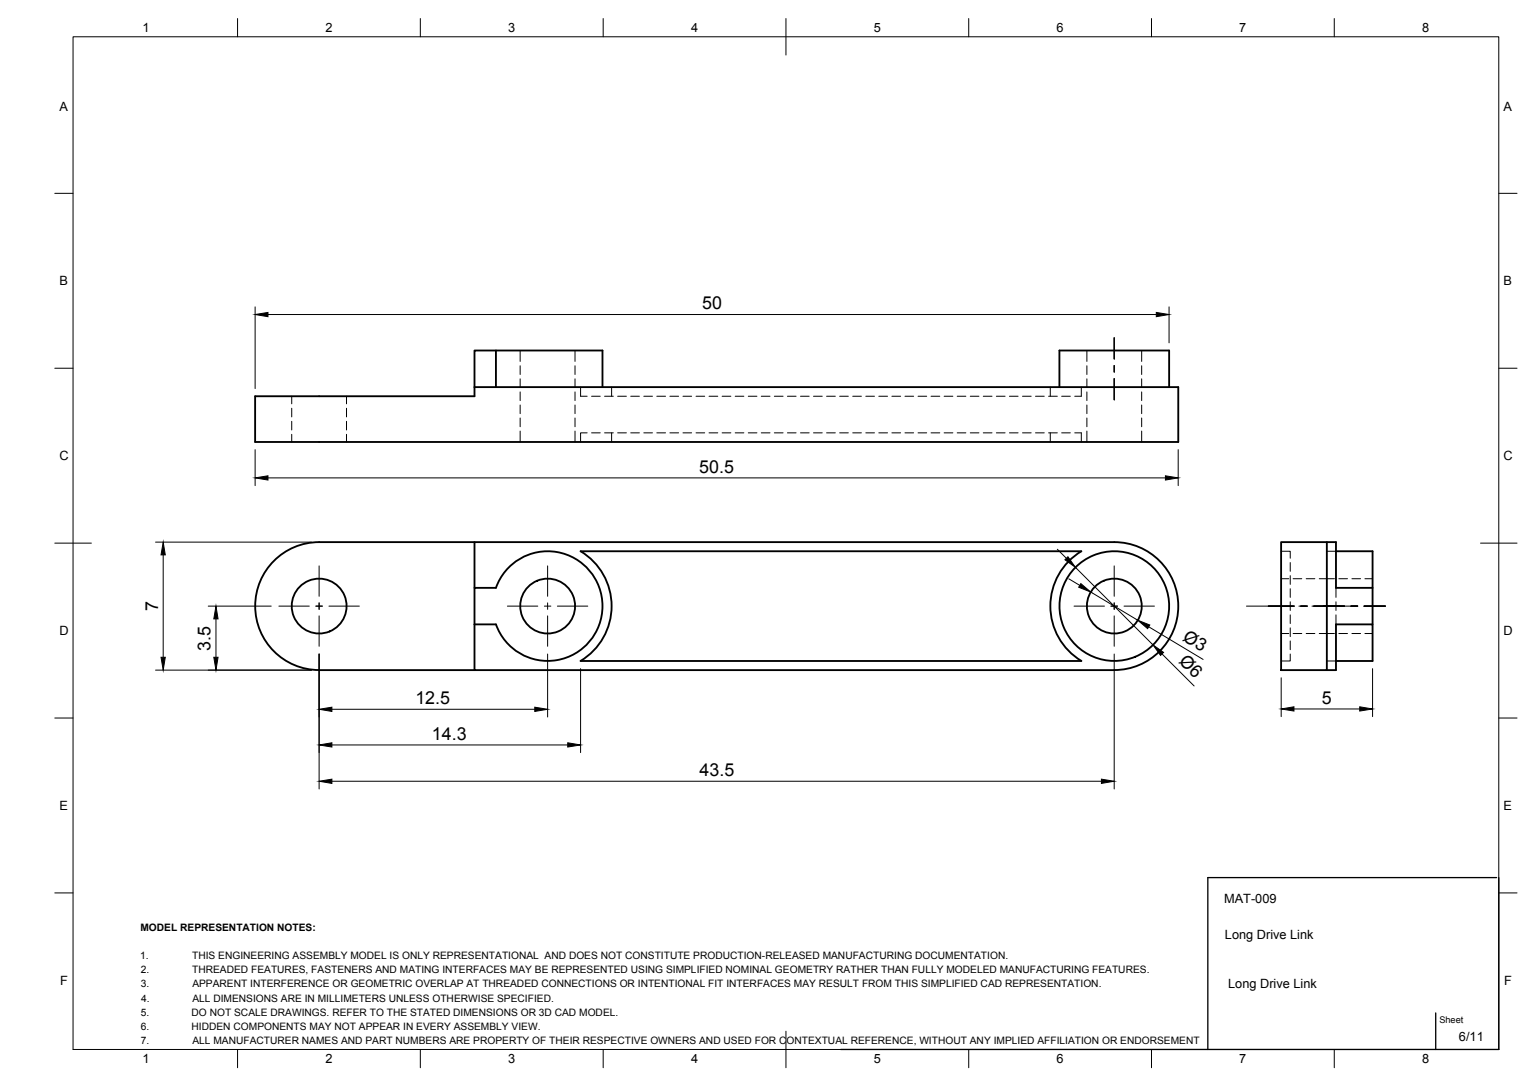
ISO-10303-21;
HEADER;
/* Generated by software containing ST-Developer
 * from STEP Tools, Inc. (www.steptools.com) 
 */

FILE_DESCRIPTION(
/* description */ ('STEP AP214'),
/* implementation_level */ '2;1');

FILE_NAME(
/* name */ 'Long Drive Link.step',
/* time_stamp */ '2026-11-14T05:43:09-08:00',
/* author */ (''),
/* organization */ (''),
/* preprocessor_version */ 'ST-DEVELOPER v20.2',
/* originating_system */ 'Autodesk Translation Framework v15.17.0.0',
/* authorisation */ '');

FILE_SCHEMA (('AUTOMOTIVE_DESIGN { 1 0 10303 214 3 1 1 }'));
ENDSEC;

DATA;
#10=MECHANICAL_DESIGN_GEOMETRIC_PRESENTATION_REPRESENTATION('',(#148),#11933);
#130=SHAPE_REPRESENTATION_RELATIONSHIP('SRR','None',#11990,#139);
#139=ADVANCED_BREP_SHAPE_REPRESENTATION('',(#157),#11926);
#148=STYLED_ITEM('',(#12043),#157);
#157=MANIFOLD_SOLID_BREP('Body1',#6645);
#183=FACE_BOUND('',#748,.T.);
#184=FACE_BOUND('',#750,.T.);
#185=FACE_BOUND('',#751,.T.);
#186=FACE_BOUND('',#753,.T.);
#187=FACE_BOUND('',#754,.T.);
#188=FACE_BOUND('',#755,.T.);
#189=FACE_BOUND('',#756,.T.);
#190=FACE_BOUND('',#773,.T.);
#191=FACE_BOUND('',#775,.T.);
#235=PLANE('',#6871);
#236=PLANE('',#6872);
#237=PLANE('',#6876);
#238=PLANE('',#6879);
#239=PLANE('',#6881);
#240=PLANE('',#6884);
#241=PLANE('',#6885);
#242=PLANE('',#6886);
#243=PLANE('',#6887);
#244=PLANE('',#6890);
#245=PLANE('',#6891);
#246=PLANE('',#6892);
#247=PLANE('',#6895);
#248=PLANE('',#6896);
#249=PLANE('',#6897);
#250=PLANE('',#6898);
#367=FACE_OUTER_BOUND('',#740,.T.);
#368=FACE_OUTER_BOUND('',#741,.T.);
#369=FACE_OUTER_BOUND('',#742,.T.);
#370=FACE_OUTER_BOUND('',#743,.T.);
#371=FACE_OUTER_BOUND('',#744,.T.);
#372=FACE_OUTER_BOUND('',#745,.T.);
#373=FACE_OUTER_BOUND('',#746,.T.);
#374=FACE_OUTER_BOUND('',#747,.T.);
#375=FACE_OUTER_BOUND('',#749,.T.);
#376=FACE_OUTER_BOUND('',#752,.T.);
#377=FACE_OUTER_BOUND('',#757,.T.);
#378=FACE_OUTER_BOUND('',#758,.T.);
#379=FACE_OUTER_BOUND('',#759,.T.);
#380=FACE_OUTER_BOUND('',#760,.T.);
#381=FACE_OUTER_BOUND('',#761,.T.);
#382=FACE_OUTER_BOUND('',#762,.T.);
#383=FACE_OUTER_BOUND('',#763,.T.);
#384=FACE_OUTER_BOUND('',#764,.T.);
#385=FACE_OUTER_BOUND('',#765,.T.);
#386=FACE_OUTER_BOUND('',#766,.T.);
#387=FACE_OUTER_BOUND('',#767,.T.);
#388=FACE_OUTER_BOUND('',#768,.T.);
#389=FACE_OUTER_BOUND('',#769,.T.);
#390=FACE_OUTER_BOUND('',#770,.T.);
#391=FACE_OUTER_BOUND('',#771,.T.);
#392=FACE_OUTER_BOUND('',#772,.T.);
#393=FACE_OUTER_BOUND('',#774,.T.);
#740=EDGE_LOOP('',(#4354,#4355,#4356,#4357));
#741=EDGE_LOOP('',(#4358,#4359,#4360,#4361));
#742=EDGE_LOOP('',(#4362,#4363,#4364,#4365));
#743=EDGE_LOOP('',(#4366,#4367,#4368,#4369));
#744=EDGE_LOOP('',(#4370,#4371,#4372,#4373));
#745=EDGE_LOOP('',(#4374,#4375,#4376,#4377));
#746=EDGE_LOOP('',(#4378,#4379,#4380,#4381));
#747=EDGE_LOOP('',(#4382,#4383,#4384,#4385));
#748=EDGE_LOOP('',(#4386));
#749=EDGE_LOOP('',(#4387,#4388,#4389,#4390,#4391,#4392,#4393,#4394));
#750=EDGE_LOOP('',(#4395,#4396,#4397,#4398));
#751=EDGE_LOOP('',(#4399));
#752=EDGE_LOOP('',(#4400,#4401,#4402,#4403));
#753=EDGE_LOOP('',(#4404));
#754=EDGE_LOOP('',(#4405,#4406,#4407,#4408));
#755=EDGE_LOOP('',(#4409));
#756=EDGE_LOOP('',(#4410));
#757=EDGE_LOOP('',(#4411,#4412,#4413,#4414,#4415,#4416));
#758=EDGE_LOOP('',(#4417,#4418,#4419,#4420));
#759=EDGE_LOOP('',(#4421,#4422,#4423,#4424,#4425,#4426));
#760=EDGE_LOOP('',(#4427,#4428,#4429,#4430));
#761=EDGE_LOOP('',(#4431,#4432,#4433,#4434));
#762=EDGE_LOOP('',(#4435,#4436,#4437,#4438));
#763=EDGE_LOOP('',(#4439,#4440,#4441,#4442));
#764=EDGE_LOOP('',(#4443,#4444,#4445,#4446));
#765=EDGE_LOOP('',(#4447,#4448,#4449,#4450));
#766=EDGE_LOOP('',(#4451,#4452,#4453,#4454));
#767=EDGE_LOOP('',(#4455,#4456,#4457,#4458));
#768=EDGE_LOOP('',(#4459,#4460,#4461,#4462));
#769=EDGE_LOOP('',(#4463,#4464,#4465,#4466));
#770=EDGE_LOOP('',(#4467,#4468,#4469,#4470));
#771=EDGE_LOOP('',(#4471,#4472,#4473,#4474,#4475,#4476,#4477,#4478));
#772=EDGE_LOOP('',(#4479,#4480,#4481,#4482));
#773=EDGE_LOOP('',(#4483));
#774=EDGE_LOOP('',(#4484));
#775=EDGE_LOOP('',(#4485));
#1147=LINE('',#10165,#1609);
#1148=LINE('',#10172,#1610);
#1149=LINE('',#10175,#1611);
#1150=LINE('',#10180,#1612);
#1151=LINE('',#10187,#1613);
#1152=LINE('',#10190,#1614);
#1153=LINE('',#10196,#1615);
#1154=LINE('',#10199,#1616);
#1155=LINE('',#10204,#1617);
#1156=LINE('',#10210,#1618);
#1157=LINE('',#10214,#1619);
#1158=LINE('',#10216,#1620);
#1159=LINE('',#10217,#1621);
#1160=LINE('',#10223,#1622);
#1161=LINE('',#10225,#1623);
#1162=LINE('',#10227,#1624);
#1163=LINE('',#10231,#1625);
#1164=LINE('',#10233,#1626);
#1165=LINE('',#10234,#1627);
#1166=LINE('',#10238,#1628);
#1167=LINE('',#10239,#1629);
#1168=LINE('',#10242,#1630);
#1169=LINE('',#10244,#1631);
#1170=LINE('',#10247,#1632);
#1171=LINE('',#10250,#1633);
#1172=LINE('',#10252,#1634);
#1173=LINE('',#10253,#1635);
#1174=LINE('',#10255,#1636);
#1175=LINE('',#10257,#1637);
#1176=LINE('',#10260,#1638);
#1177=LINE('',#10263,#1639);
#1178=LINE('',#10265,#1640);
#1179=LINE('',#10267,#1641);
#1180=LINE('',#10271,#1642);
#1181=LINE('',#10272,#1643);
#1182=LINE('',#10276,#1644);
#1183=LINE('',#10278,#1645);
#1184=LINE('',#10282,#1646);
#1185=LINE('',#10284,#1647);
#1186=LINE('',#10285,#1648);
#1187=LINE('',#10288,#1649);
#1188=LINE('',#10292,#1650);
#1189=LINE('',#10293,#1651);
#1190=LINE('',#10295,#1652);
#1609=VECTOR('',#7925,1.5);
#1610=VECTOR('',#7932,1000.);
#1611=VECTOR('',#7935,1000.);
#1612=VECTOR('',#7940,3.);
#1613=VECTOR('',#7947,1000.);
#1614=VECTOR('',#7950,1000.);
#1615=VECTOR('',#7955,1000.);
#1616=VECTOR('',#7958,1000.);
#1617=VECTOR('',#7963,1.5);
#1618=VECTOR('',#7970,1.5);
#1619=VECTOR('',#7975,1000.);
#1620=VECTOR('',#7976,1000.);
#1621=VECTOR('',#7977,1000.);
#1622=VECTOR('',#7982,1000.);
#1623=VECTOR('',#7983,1000.);
#1624=VECTOR('',#7984,1000.);
#1625=VECTOR('',#7987,1000.);
#1626=VECTOR('',#7988,1000.);
#1627=VECTOR('',#7989,1000.);
#1628=VECTOR('',#7992,1000.);
#1629=VECTOR('',#7993,1000.);
#1630=VECTOR('',#7996,1000.);
#1631=VECTOR('',#7997,1000.);
#1632=VECTOR('',#8000,1000.);
#1633=VECTOR('',#8003,1000.);
#1634=VECTOR('',#8006,1000.);
#1635=VECTOR('',#8007,1000.);
#1636=VECTOR('',#8010,1000.);
#1637=VECTOR('',#8013,1000.);
#1638=VECTOR('',#8016,1000.);
#1639=VECTOR('',#8019,1000.);
#1640=VECTOR('',#8022,1000.);
#1641=VECTOR('',#8025,1000.);
#1642=VECTOR('',#8030,1000.);
#1643=VECTOR('',#8031,1000.);
#1644=VECTOR('',#8036,1000.);
#1645=VECTOR('',#8039,1000.);
#1646=VECTOR('',#8044,1000.);
#1647=VECTOR('',#8045,1000.);
#1648=VECTOR('',#8046,1000.);
#1649=VECTOR('',#8049,1000.);
#1650=VECTOR('',#8054,1000.);
#1651=VECTOR('',#8055,1000.);
#1652=VECTOR('',#8058,1000.);
#2042=CIRCLE('',#6851,1.5);
#2043=CIRCLE('',#6852,1.5);
#2044=CIRCLE('',#6854,3.5);
#2045=CIRCLE('',#6855,3.5);
#2046=CIRCLE('',#6857,3.);
#2047=CIRCLE('',#6858,3.);
#2048=CIRCLE('',#6860,3.5);
#2049=CIRCLE('',#6861,3.5);
#2050=CIRCLE('',#6863,3.5);
#2051=CIRCLE('',#6864,3.5);
#2052=CIRCLE('',#6866,1.5);
#2053=CIRCLE('',#6867,1.5);
#2054=CIRCLE('',#6869,1.5);
#2055=CIRCLE('',#6870,1.5);
#2056=CIRCLE('',#6873,3.);
#2057=CIRCLE('',#6874,3.5);
#2058=CIRCLE('',#6875,3.5);
#2059=CIRCLE('',#6877,3.5);
#2060=CIRCLE('',#6878,3.5);
#2061=CIRCLE('',#6883,3.5);
#2062=CIRCLE('',#6889,3.5);
#2063=CIRCLE('',#6894,3.);
#2581=VERTEX_POINT('',#10162);
#2582=VERTEX_POINT('',#10164);
#2583=VERTEX_POINT('',#10168);
#2584=VERTEX_POINT('',#10169);
#2585=VERTEX_POINT('',#10171);
#2586=VERTEX_POINT('',#10173);
#2587=VERTEX_POINT('',#10177);
#2588=VERTEX_POINT('',#10179);
#2589=VERTEX_POINT('',#10183);
#2590=VERTEX_POINT('',#10184);
#2591=VERTEX_POINT('',#10186);
#2592=VERTEX_POINT('',#10188);
#2593=VERTEX_POINT('',#10192);
#2594=VERTEX_POINT('',#10193);
#2595=VERTEX_POINT('',#10195);
#2596=VERTEX_POINT('',#10197);
#2597=VERTEX_POINT('',#10201);
#2598=VERTEX_POINT('',#10203);
#2599=VERTEX_POINT('',#10207);
#2600=VERTEX_POINT('',#10209);
#2601=VERTEX_POINT('',#10213);
#2602=VERTEX_POINT('',#10215);
#2603=VERTEX_POINT('',#10219);
#2604=VERTEX_POINT('',#10220);
#2605=VERTEX_POINT('',#10222);
#2606=VERTEX_POINT('',#10224);
#2607=VERTEX_POINT('',#10226);
#2608=VERTEX_POINT('',#10228);
#2609=VERTEX_POINT('',#10230);
#2610=VERTEX_POINT('',#10232);
#2611=VERTEX_POINT('',#10235);
#2612=VERTEX_POINT('',#10236);
#2613=VERTEX_POINT('',#10241);
#2614=VERTEX_POINT('',#10243);
#2615=VERTEX_POINT('',#10246);
#2616=VERTEX_POINT('',#10248);
#2617=VERTEX_POINT('',#10259);
#2618=VERTEX_POINT('',#10261);
#2619=VERTEX_POINT('',#10270);
#2620=VERTEX_POINT('',#10274);
#2621=VERTEX_POINT('',#10281);
#2622=VERTEX_POINT('',#10283);
#2623=VERTEX_POINT('',#10287);
#2624=VERTEX_POINT('',#10291);
#3266=EDGE_CURVE('',#2581,#2581,#2042,.T.);
#3267=EDGE_CURVE('',#2581,#2582,#1147,.T.);
#3268=EDGE_CURVE('',#2582,#2582,#2043,.T.);
#3269=EDGE_CURVE('',#2583,#2584,#2044,.T.);
#3270=EDGE_CURVE('',#2583,#2585,#1148,.T.);
#3271=EDGE_CURVE('',#2585,#2586,#2045,.T.);
#3272=EDGE_CURVE('',#2584,#2586,#1149,.T.);
#3273=EDGE_CURVE('',#2587,#2587,#2046,.T.);
#3274=EDGE_CURVE('',#2587,#2588,#1150,.T.);
#3275=EDGE_CURVE('',#2588,#2588,#2047,.T.);
#3276=EDGE_CURVE('',#2589,#2590,#2048,.T.);
#3277=EDGE_CURVE('',#2590,#2591,#1151,.T.);
#3278=EDGE_CURVE('',#2592,#2591,#2049,.T.);
#3279=EDGE_CURVE('',#2589,#2592,#1152,.T.);
#3280=EDGE_CURVE('',#2593,#2594,#2050,.T.);
#3281=EDGE_CURVE('',#2593,#2595,#1153,.T.);
#3282=EDGE_CURVE('',#2595,#2596,#2051,.T.);
#3283=EDGE_CURVE('',#2594,#2596,#1154,.T.);
#3284=EDGE_CURVE('',#2597,#2597,#2052,.T.);
#3285=EDGE_CURVE('',#2597,#2598,#1155,.T.);
#3286=EDGE_CURVE('',#2598,#2598,#2053,.T.);
#3287=EDGE_CURVE('',#2599,#2599,#2054,.T.);
#3288=EDGE_CURVE('',#2599,#2600,#1156,.T.);
#3289=EDGE_CURVE('',#2600,#2600,#2055,.T.);
#3290=EDGE_CURVE('',#2584,#2601,#1157,.T.);
#3291=EDGE_CURVE('',#2602,#2601,#1158,.T.);
#3292=EDGE_CURVE('',#2602,#2583,#1159,.T.);
#3293=EDGE_CURVE('',#2603,#2604,#2056,.T.);
#3294=EDGE_CURVE('',#2603,#2605,#1160,.T.);
#3295=EDGE_CURVE('',#2605,#2606,#1161,.T.);
#3296=EDGE_CURVE('',#2606,#2607,#1162,.T.);
#3297=EDGE_CURVE('',#2607,#2608,#2057,.T.);
#3298=EDGE_CURVE('',#2608,#2609,#1163,.T.);
#3299=EDGE_CURVE('',#2609,#2610,#1164,.T.);
#3300=EDGE_CURVE('',#2604,#2610,#1165,.T.);
#3301=EDGE_CURVE('',#2611,#2612,#2058,.T.);
#3302=EDGE_CURVE('',#2596,#2611,#1166,.T.);
#3303=EDGE_CURVE('',#2612,#2595,#1167,.T.);
#3304=EDGE_CURVE('',#2586,#2613,#1168,.T.);
#3305=EDGE_CURVE('',#2614,#2585,#1169,.T.);
#3306=EDGE_CURVE('',#2613,#2614,#2059,.T.);
#3307=EDGE_CURVE('',#2591,#2615,#1170,.T.);
#3308=EDGE_CURVE('',#2615,#2616,#2060,.T.);
#3309=EDGE_CURVE('',#2616,#2592,#1171,.T.);
#3310=EDGE_CURVE('',#2607,#2613,#1172,.T.);
#3311=EDGE_CURVE('',#2606,#2601,#1173,.T.);
#3312=EDGE_CURVE('',#2608,#2614,#1174,.T.);
#3313=EDGE_CURVE('',#2609,#2602,#1175,.T.);
#3314=EDGE_CURVE('',#2617,#2612,#1176,.T.);
#3315=EDGE_CURVE('',#2618,#2617,#2061,.T.);
#3316=EDGE_CURVE('',#2618,#2611,#1177,.T.);
#3317=EDGE_CURVE('',#2594,#2618,#1178,.T.);
#3318=EDGE_CURVE('',#2617,#2593,#1179,.T.);
#3319=EDGE_CURVE('',#2590,#2619,#1180,.T.);
#3320=EDGE_CURVE('',#2619,#2615,#1181,.T.);
#3321=EDGE_CURVE('',#2619,#2620,#2062,.T.);
#3322=EDGE_CURVE('',#2620,#2616,#1182,.T.);
#3323=EDGE_CURVE('',#2620,#2589,#1183,.T.);
#3324=EDGE_CURVE('',#2621,#2603,#1184,.T.);
#3325=EDGE_CURVE('',#2621,#2622,#1185,.T.);
#3326=EDGE_CURVE('',#2622,#2605,#1186,.T.);
#3327=EDGE_CURVE('',#2623,#2604,#1187,.T.);
#3328=EDGE_CURVE('',#2621,#2623,#2063,.T.);
#3329=EDGE_CURVE('',#2624,#2610,#1188,.T.);
#3330=EDGE_CURVE('',#2623,#2624,#1189,.T.);
#3331=EDGE_CURVE('',#2624,#2622,#1190,.T.);
#4354=ORIENTED_EDGE('',*,*,#3266,.T.);
#4355=ORIENTED_EDGE('',*,*,#3267,.T.);
#4356=ORIENTED_EDGE('',*,*,#3268,.F.);
#4357=ORIENTED_EDGE('',*,*,#3267,.F.);
#4358=ORIENTED_EDGE('',*,*,#3269,.F.);
#4359=ORIENTED_EDGE('',*,*,#3270,.T.);
#4360=ORIENTED_EDGE('',*,*,#3271,.T.);
#4361=ORIENTED_EDGE('',*,*,#3272,.F.);
#4362=ORIENTED_EDGE('',*,*,#3273,.T.);
#4363=ORIENTED_EDGE('',*,*,#3274,.T.);
#4364=ORIENTED_EDGE('',*,*,#3275,.F.);
#4365=ORIENTED_EDGE('',*,*,#3274,.F.);
#4366=ORIENTED_EDGE('',*,*,#3276,.T.);
#4367=ORIENTED_EDGE('',*,*,#3277,.T.);
#4368=ORIENTED_EDGE('',*,*,#3278,.F.);
#4369=ORIENTED_EDGE('',*,*,#3279,.F.);
#4370=ORIENTED_EDGE('',*,*,#3280,.F.);
#4371=ORIENTED_EDGE('',*,*,#3281,.T.);
#4372=ORIENTED_EDGE('',*,*,#3282,.T.);
#4373=ORIENTED_EDGE('',*,*,#3283,.F.);
#4374=ORIENTED_EDGE('',*,*,#3284,.F.);
#4375=ORIENTED_EDGE('',*,*,#3285,.T.);
#4376=ORIENTED_EDGE('',*,*,#3286,.F.);
#4377=ORIENTED_EDGE('',*,*,#3285,.F.);
#4378=ORIENTED_EDGE('',*,*,#3287,.F.);
#4379=ORIENTED_EDGE('',*,*,#3288,.T.);
#4380=ORIENTED_EDGE('',*,*,#3289,.F.);
#4381=ORIENTED_EDGE('',*,*,#3288,.F.);
#4382=ORIENTED_EDGE('',*,*,#3290,.T.);
#4383=ORIENTED_EDGE('',*,*,#3291,.F.);
#4384=ORIENTED_EDGE('',*,*,#3292,.T.);
#4385=ORIENTED_EDGE('',*,*,#3269,.T.);
#4386=ORIENTED_EDGE('',*,*,#3266,.F.);
#4387=ORIENTED_EDGE('',*,*,#3293,.F.);
#4388=ORIENTED_EDGE('',*,*,#3294,.T.);
#4389=ORIENTED_EDGE('',*,*,#3295,.T.);
#4390=ORIENTED_EDGE('',*,*,#3296,.T.);
#4391=ORIENTED_EDGE('',*,*,#3297,.T.);
#4392=ORIENTED_EDGE('',*,*,#3298,.T.);
#4393=ORIENTED_EDGE('',*,*,#3299,.T.);
#4394=ORIENTED_EDGE('',*,*,#3300,.F.);
#4395=ORIENTED_EDGE('',*,*,#3301,.F.);
#4396=ORIENTED_EDGE('',*,*,#3302,.F.);
#4397=ORIENTED_EDGE('',*,*,#3282,.F.);
#4398=ORIENTED_EDGE('',*,*,#3303,.F.);
#4399=ORIENTED_EDGE('',*,*,#3273,.F.);
#4400=ORIENTED_EDGE('',*,*,#3304,.F.);
#4401=ORIENTED_EDGE('',*,*,#3271,.F.);
#4402=ORIENTED_EDGE('',*,*,#3305,.F.);
#4403=ORIENTED_EDGE('',*,*,#3306,.F.);
#4404=ORIENTED_EDGE('',*,*,#3289,.T.);
#4405=ORIENTED_EDGE('',*,*,#3278,.T.);
#4406=ORIENTED_EDGE('',*,*,#3307,.T.);
#4407=ORIENTED_EDGE('',*,*,#3308,.T.);
#4408=ORIENTED_EDGE('',*,*,#3309,.T.);
#4409=ORIENTED_EDGE('',*,*,#3268,.T.);
#4410=ORIENTED_EDGE('',*,*,#3286,.T.);
#4411=ORIENTED_EDGE('',*,*,#3304,.T.);
#4412=ORIENTED_EDGE('',*,*,#3310,.F.);
#4413=ORIENTED_EDGE('',*,*,#3296,.F.);
#4414=ORIENTED_EDGE('',*,*,#3311,.T.);
#4415=ORIENTED_EDGE('',*,*,#3290,.F.);
#4416=ORIENTED_EDGE('',*,*,#3272,.T.);
#4417=ORIENTED_EDGE('',*,*,#3306,.T.);
#4418=ORIENTED_EDGE('',*,*,#3312,.F.);
#4419=ORIENTED_EDGE('',*,*,#3297,.F.);
#4420=ORIENTED_EDGE('',*,*,#3310,.T.);
#4421=ORIENTED_EDGE('',*,*,#3305,.T.);
#4422=ORIENTED_EDGE('',*,*,#3270,.F.);
#4423=ORIENTED_EDGE('',*,*,#3292,.F.);
#4424=ORIENTED_EDGE('',*,*,#3313,.F.);
#4425=ORIENTED_EDGE('',*,*,#3298,.F.);
#4426=ORIENTED_EDGE('',*,*,#3312,.T.);
#4427=ORIENTED_EDGE('',*,*,#3301,.T.);
#4428=ORIENTED_EDGE('',*,*,#3314,.F.);
#4429=ORIENTED_EDGE('',*,*,#3315,.F.);
#4430=ORIENTED_EDGE('',*,*,#3316,.T.);
#4431=ORIENTED_EDGE('',*,*,#3302,.T.);
#4432=ORIENTED_EDGE('',*,*,#3316,.F.);
#4433=ORIENTED_EDGE('',*,*,#3317,.F.);
#4434=ORIENTED_EDGE('',*,*,#3283,.T.);
#4435=ORIENTED_EDGE('',*,*,#3303,.T.);
#4436=ORIENTED_EDGE('',*,*,#3281,.F.);
#4437=ORIENTED_EDGE('',*,*,#3318,.F.);
#4438=ORIENTED_EDGE('',*,*,#3314,.T.);
#4439=ORIENTED_EDGE('',*,*,#3315,.T.);
#4440=ORIENTED_EDGE('',*,*,#3318,.T.);
#4441=ORIENTED_EDGE('',*,*,#3280,.T.);
#4442=ORIENTED_EDGE('',*,*,#3317,.T.);
#4443=ORIENTED_EDGE('',*,*,#3307,.F.);
#4444=ORIENTED_EDGE('',*,*,#3277,.F.);
#4445=ORIENTED_EDGE('',*,*,#3319,.T.);
#4446=ORIENTED_EDGE('',*,*,#3320,.T.);
#4447=ORIENTED_EDGE('',*,*,#3308,.F.);
#4448=ORIENTED_EDGE('',*,*,#3320,.F.);
#4449=ORIENTED_EDGE('',*,*,#3321,.T.);
#4450=ORIENTED_EDGE('',*,*,#3322,.T.);
#4451=ORIENTED_EDGE('',*,*,#3309,.F.);
#4452=ORIENTED_EDGE('',*,*,#3322,.F.);
#4453=ORIENTED_EDGE('',*,*,#3323,.T.);
#4454=ORIENTED_EDGE('',*,*,#3279,.T.);
#4455=ORIENTED_EDGE('',*,*,#3276,.F.);
#4456=ORIENTED_EDGE('',*,*,#3323,.F.);
#4457=ORIENTED_EDGE('',*,*,#3321,.F.);
#4458=ORIENTED_EDGE('',*,*,#3319,.F.);
#4459=ORIENTED_EDGE('',*,*,#3294,.F.);
#4460=ORIENTED_EDGE('',*,*,#3324,.F.);
#4461=ORIENTED_EDGE('',*,*,#3325,.T.);
#4462=ORIENTED_EDGE('',*,*,#3326,.T.);
#4463=ORIENTED_EDGE('',*,*,#3293,.T.);
#4464=ORIENTED_EDGE('',*,*,#3327,.F.);
#4465=ORIENTED_EDGE('',*,*,#3328,.F.);
#4466=ORIENTED_EDGE('',*,*,#3324,.T.);
#4467=ORIENTED_EDGE('',*,*,#3300,.T.);
#4468=ORIENTED_EDGE('',*,*,#3329,.F.);
#4469=ORIENTED_EDGE('',*,*,#3330,.F.);
#4470=ORIENTED_EDGE('',*,*,#3327,.T.);
#4471=ORIENTED_EDGE('',*,*,#3329,.T.);
#4472=ORIENTED_EDGE('',*,*,#3299,.F.);
#4473=ORIENTED_EDGE('',*,*,#3313,.T.);
#4474=ORIENTED_EDGE('',*,*,#3291,.T.);
#4475=ORIENTED_EDGE('',*,*,#3311,.F.);
#4476=ORIENTED_EDGE('',*,*,#3295,.F.);
#4477=ORIENTED_EDGE('',*,*,#3326,.F.);
#4478=ORIENTED_EDGE('',*,*,#3331,.F.);
#4479=ORIENTED_EDGE('',*,*,#3325,.F.);
#4480=ORIENTED_EDGE('',*,*,#3328,.T.);
#4481=ORIENTED_EDGE('',*,*,#3330,.T.);
#4482=ORIENTED_EDGE('',*,*,#3331,.T.);
#4483=ORIENTED_EDGE('',*,*,#3287,.T.);
#4484=ORIENTED_EDGE('',*,*,#3275,.T.);
#4485=ORIENTED_EDGE('',*,*,#3284,.T.);
#6068=CYLINDRICAL_SURFACE('',#6850,1.5);
#6069=CYLINDRICAL_SURFACE('',#6853,3.5);
#6070=CYLINDRICAL_SURFACE('',#6856,3.);
#6071=CYLINDRICAL_SURFACE('',#6859,3.5);
#6072=CYLINDRICAL_SURFACE('',#6862,3.5);
#6073=CYLINDRICAL_SURFACE('',#6865,1.5);
#6074=CYLINDRICAL_SURFACE('',#6868,1.5);
#6075=CYLINDRICAL_SURFACE('',#6880,3.5);
#6076=CYLINDRICAL_SURFACE('',#6882,3.5);
#6077=CYLINDRICAL_SURFACE('',#6888,3.5);
#6078=CYLINDRICAL_SURFACE('',#6893,3.);
#6337=ADVANCED_FACE('',(#367),#6068,.F.);
#6338=ADVANCED_FACE('',(#368),#6069,.T.);
#6339=ADVANCED_FACE('',(#369),#6070,.T.);
#6340=ADVANCED_FACE('',(#370),#6071,.T.);
#6341=ADVANCED_FACE('',(#371),#6072,.T.);
#6342=ADVANCED_FACE('',(#372),#6073,.F.);
#6343=ADVANCED_FACE('',(#373),#6074,.F.);
#6344=ADVANCED_FACE('',(#374,#183),#235,.T.);
#6345=ADVANCED_FACE('',(#375,#184,#185),#236,.T.);
#6346=ADVANCED_FACE('',(#376,#186,#187,#188,#189),#237,.F.);
#6347=ADVANCED_FACE('',(#377),#238,.F.);
#6348=ADVANCED_FACE('',(#378),#6075,.T.);
#6349=ADVANCED_FACE('',(#379),#239,.F.);
#6350=ADVANCED_FACE('',(#380),#6076,.T.);
#6351=ADVANCED_FACE('',(#381),#240,.F.);
#6352=ADVANCED_FACE('',(#382),#241,.F.);
#6353=ADVANCED_FACE('',(#383),#242,.T.);
#6354=ADVANCED_FACE('',(#384),#243,.T.);
#6355=ADVANCED_FACE('',(#385),#6077,.T.);
#6356=ADVANCED_FACE('',(#386),#244,.T.);
#6357=ADVANCED_FACE('',(#387),#245,.T.);
#6358=ADVANCED_FACE('',(#388),#246,.T.);
#6359=ADVANCED_FACE('',(#389),#6078,.T.);
#6360=ADVANCED_FACE('',(#390),#247,.F.);
#6361=ADVANCED_FACE('',(#391),#248,.F.);
#6362=ADVANCED_FACE('',(#392,#190),#249,.T.);
#6363=ADVANCED_FACE('',(#393,#191),#250,.T.);
#6645=CLOSED_SHELL('',(#6337,#6338,#6339,#6340,#6341,#6342,#6343,#6344,
#6345,#6346,#6347,#6348,#6349,#6350,#6351,#6352,#6353,#6354,#6355,#6356,
#6357,#6358,#6359,#6360,#6361,#6362,#6363));
#6849=AXIS2_PLACEMENT_3D('',#10160,#7919,#7920);
#6850=AXIS2_PLACEMENT_3D('',#10161,#7921,#7922);
#6851=AXIS2_PLACEMENT_3D('',#10163,#7923,#7924);
#6852=AXIS2_PLACEMENT_3D('',#10166,#7926,#7927);
#6853=AXIS2_PLACEMENT_3D('',#10167,#7928,#7929);
#6854=AXIS2_PLACEMENT_3D('',#10170,#7930,#7931);
#6855=AXIS2_PLACEMENT_3D('',#10174,#7933,#7934);
#6856=AXIS2_PLACEMENT_3D('',#10176,#7936,#7937);
#6857=AXIS2_PLACEMENT_3D('',#10178,#7938,#7939);
#6858=AXIS2_PLACEMENT_3D('',#10181,#7941,#7942);
#6859=AXIS2_PLACEMENT_3D('',#10182,#7943,#7944);
#6860=AXIS2_PLACEMENT_3D('',#10185,#7945,#7946);
#6861=AXIS2_PLACEMENT_3D('',#10189,#7948,#7949);
#6862=AXIS2_PLACEMENT_3D('',#10191,#7951,#7952);
#6863=AXIS2_PLACEMENT_3D('',#10194,#7953,#7954);
#6864=AXIS2_PLACEMENT_3D('',#10198,#7956,#7957);
#6865=AXIS2_PLACEMENT_3D('',#10200,#7959,#7960);
#6866=AXIS2_PLACEMENT_3D('',#10202,#7961,#7962);
#6867=AXIS2_PLACEMENT_3D('',#10205,#7964,#7965);
#6868=AXIS2_PLACEMENT_3D('',#10206,#7966,#7967);
#6869=AXIS2_PLACEMENT_3D('',#10208,#7968,#7969);
#6870=AXIS2_PLACEMENT_3D('',#10211,#7971,#7972);
#6871=AXIS2_PLACEMENT_3D('',#10212,#7973,#7974);
#6872=AXIS2_PLACEMENT_3D('',#10218,#7978,#7979);
#6873=AXIS2_PLACEMENT_3D('',#10221,#7980,#7981);
#6874=AXIS2_PLACEMENT_3D('',#10229,#7985,#7986);
#6875=AXIS2_PLACEMENT_3D('',#10237,#7990,#7991);
#6876=AXIS2_PLACEMENT_3D('',#10240,#7994,#7995);
#6877=AXIS2_PLACEMENT_3D('',#10245,#7998,#7999);
#6878=AXIS2_PLACEMENT_3D('',#10249,#8001,#8002);
#6879=AXIS2_PLACEMENT_3D('',#10251,#8004,#8005);
#6880=AXIS2_PLACEMENT_3D('',#10254,#8008,#8009);
#6881=AXIS2_PLACEMENT_3D('',#10256,#8011,#8012);
#6882=AXIS2_PLACEMENT_3D('',#10258,#8014,#8015);
#6883=AXIS2_PLACEMENT_3D('',#10262,#8017,#8018);
#6884=AXIS2_PLACEMENT_3D('',#10264,#8020,#8021);
#6885=AXIS2_PLACEMENT_3D('',#10266,#8023,#8024);
#6886=AXIS2_PLACEMENT_3D('',#10268,#8026,#8027);
#6887=AXIS2_PLACEMENT_3D('',#10269,#8028,#8029);
#6888=AXIS2_PLACEMENT_3D('',#10273,#8032,#8033);
#6889=AXIS2_PLACEMENT_3D('',#10275,#8034,#8035);
#6890=AXIS2_PLACEMENT_3D('',#10277,#8037,#8038);
#6891=AXIS2_PLACEMENT_3D('',#10279,#8040,#8041);
#6892=AXIS2_PLACEMENT_3D('',#10280,#8042,#8043);
#6893=AXIS2_PLACEMENT_3D('',#10286,#8047,#8048);
#6894=AXIS2_PLACEMENT_3D('',#10289,#8050,#8051);
#6895=AXIS2_PLACEMENT_3D('',#10290,#8052,#8053);
#6896=AXIS2_PLACEMENT_3D('',#10294,#8056,#8057);
#6897=AXIS2_PLACEMENT_3D('',#10296,#8059,#8060);
#6898=AXIS2_PLACEMENT_3D('',#10297,#8061,#8062);
#7919=DIRECTION('axis',(0.,0.,1.));
#7920=DIRECTION('refdir',(1.,0.,0.));
#7921=DIRECTION('center_axis',(0.,0.,-1.));
#7922=DIRECTION('ref_axis',(-1.,0.,0.));
#7923=DIRECTION('center_axis',(0.,0.,1.));
#7924=DIRECTION('ref_axis',(1.,0.,0.));
#7925=DIRECTION('',(0.,0.,-1.));
#7926=DIRECTION('center_axis',(0.,0.,1.));
#7927=DIRECTION('ref_axis',(1.,0.,0.));
#7928=DIRECTION('center_axis',(0.,0.,-1.));
#7929=DIRECTION('ref_axis',(-1.,0.,0.));
#7930=DIRECTION('center_axis',(0.,0.,1.));
#7931=DIRECTION('ref_axis',(1.,0.,0.));
#7932=DIRECTION('',(0.,0.,-1.));
#7933=DIRECTION('center_axis',(0.,0.,1.));
#7934=DIRECTION('ref_axis',(1.,0.,0.));
#7935=DIRECTION('',(0.,0.,-1.));
#7936=DIRECTION('center_axis',(0.,0.,-1.));
#7937=DIRECTION('ref_axis',(-1.,0.,0.));
#7938=DIRECTION('center_axis',(0.,0.,1.));
#7939=DIRECTION('ref_axis',(1.,0.,0.));
#7940=DIRECTION('',(0.,0.,1.));
#7941=DIRECTION('center_axis',(0.,0.,1.));
#7942=DIRECTION('ref_axis',(1.,0.,0.));
#7943=DIRECTION('center_axis',(0.,0.,-1.));
#7944=DIRECTION('ref_axis',(-1.,0.,0.));
#7945=DIRECTION('center_axis',(0.,0.,-1.));
#7946=DIRECTION('ref_axis',(1.,0.,0.));
#7947=DIRECTION('',(0.,0.,-1.));
#7948=DIRECTION('center_axis',(0.,0.,-1.));
#7949=DIRECTION('ref_axis',(1.,0.,0.));
#7950=DIRECTION('',(0.,0.,-1.));
#7951=DIRECTION('center_axis',(0.,0.,1.));
#7952=DIRECTION('ref_axis',(1.,0.,0.));
#7953=DIRECTION('center_axis',(0.,0.,-1.));
#7954=DIRECTION('ref_axis',(1.,0.,0.));
#7955=DIRECTION('',(0.,0.,1.));
#7956=DIRECTION('center_axis',(0.,0.,-1.));
#7957=DIRECTION('ref_axis',(1.,0.,0.));
#7958=DIRECTION('',(0.,0.,1.));
#7959=DIRECTION('center_axis',(0.,0.,-1.));
#7960=DIRECTION('ref_axis',(-1.,0.,0.));
#7961=DIRECTION('center_axis',(0.,0.,-1.));
#7962=DIRECTION('ref_axis',(1.,0.,0.));
#7963=DIRECTION('',(0.,0.,-1.));
#7964=DIRECTION('center_axis',(0.,0.,1.));
#7965=DIRECTION('ref_axis',(1.,0.,0.));
#7966=DIRECTION('center_axis',(0.,0.,-1.));
#7967=DIRECTION('ref_axis',(-1.,0.,0.));
#7968=DIRECTION('center_axis',(0.,0.,-1.));
#7969=DIRECTION('ref_axis',(1.,0.,0.));
#7970=DIRECTION('',(0.,0.,-1.));
#7971=DIRECTION('center_axis',(0.,0.,1.));
#7972=DIRECTION('ref_axis',(1.,0.,0.));
#7973=DIRECTION('center_axis',(0.,0.,1.));
#7974=DIRECTION('ref_axis',(1.,0.,0.));
#7975=DIRECTION('',(1.,0.,0.));
#7976=DIRECTION('',(0.,-1.,0.));
#7977=DIRECTION('',(-1.,-1.38777878078145E-16,0.));
#7978=DIRECTION('center_axis',(0.,0.,1.));
#7979=DIRECTION('ref_axis',(1.,0.,0.));
#7980=DIRECTION('center_axis',(0.,0.,1.));
#7981=DIRECTION('ref_axis',(1.,0.,0.));
#7982=DIRECTION('',(-1.,0.,0.));
#7983=DIRECTION('',(0.,-1.,0.));
#7984=DIRECTION('',(1.,-1.39897054514259E-17,0.));
#7985=DIRECTION('center_axis',(0.,0.,1.));
#7986=DIRECTION('ref_axis',(1.,0.,0.));
#7987=DIRECTION('',(-1.,0.,0.));
#7988=DIRECTION('',(0.,-1.,0.));
#7989=DIRECTION('',(-1.,0.,0.));
#7990=DIRECTION('center_axis',(0.,0.,-1.));
#7991=DIRECTION('ref_axis',(1.,0.,0.));
#7992=DIRECTION('',(1.,3.16619526353726E-17,0.));
#7993=DIRECTION('',(-1.,3.16619526353726E-17,0.));
#7994=DIRECTION('center_axis',(0.,0.,1.));
#7995=DIRECTION('ref_axis',(1.,0.,0.));
#7996=DIRECTION('',(1.,-1.39897054514259E-17,0.));
#7997=DIRECTION('',(-1.,0.,0.));
#7998=DIRECTION('center_axis',(0.,0.,1.));
#7999=DIRECTION('ref_axis',(1.,0.,0.));
#8000=DIRECTION('',(-1.,3.16619526353726E-17,0.));
#8001=DIRECTION('center_axis',(0.,0.,-1.));
#8002=DIRECTION('ref_axis',(1.,0.,0.));
#8003=DIRECTION('',(1.,3.16619526353726E-17,0.));
#8004=DIRECTION('center_axis',(1.39897054514259E-17,1.,0.));
#8005=DIRECTION('ref_axis',(-1.,1.39897054514259E-17,0.));
#8006=DIRECTION('',(0.,0.,-1.));
#8007=DIRECTION('',(0.,0.,-1.));
#8008=DIRECTION('center_axis',(0.,0.,-1.));
#8009=DIRECTION('ref_axis',(1.,1.22464679914735E-16,0.));
#8010=DIRECTION('',(0.,0.,-1.));
#8011=DIRECTION('center_axis',(0.,-1.,0.));
#8012=DIRECTION('ref_axis',(0.,0.,-1.));
#8013=DIRECTION('',(0.,0.,-1.));
#8014=DIRECTION('center_axis',(0.,0.,1.));
#8015=DIRECTION('ref_axis',(-1.,1.22464679914735E-16,0.));
#8016=DIRECTION('',(0.,0.,1.));
#8017=DIRECTION('center_axis',(0.,0.,-1.));
#8018=DIRECTION('ref_axis',(1.,0.,0.));
#8019=DIRECTION('',(0.,0.,1.));
#8020=DIRECTION('center_axis',(3.16619526353726E-17,-1.,0.));
#8021=DIRECTION('ref_axis',(1.,3.16619526353726E-17,0.));
#8022=DIRECTION('',(1.,3.16619526353726E-17,0.));
#8023=DIRECTION('center_axis',(3.16619526353726E-17,1.,0.));
#8024=DIRECTION('ref_axis',(-1.,3.16619526353726E-17,0.));
#8025=DIRECTION('',(-1.,3.16619526353726E-17,0.));
#8026=DIRECTION('center_axis',(0.,0.,1.));
#8027=DIRECTION('ref_axis',(1.,0.,0.));
#8028=DIRECTION('center_axis',(-3.16619526353726E-17,-1.,0.));
#8029=DIRECTION('ref_axis',(1.,-3.16619526353726E-17,0.));
#8030=DIRECTION('',(-1.,3.16619526353726E-17,0.));
#8031=DIRECTION('',(0.,0.,-1.));
#8032=DIRECTION('center_axis',(0.,0.,-1.));
#8033=DIRECTION('ref_axis',(1.,1.22464679914735E-16,0.));
#8034=DIRECTION('center_axis',(0.,0.,-1.));
#8035=DIRECTION('ref_axis',(1.,0.,0.));
#8036=DIRECTION('',(0.,0.,-1.));
#8037=DIRECTION('center_axis',(-3.16619526353726E-17,1.,0.));
#8038=DIRECTION('ref_axis',(-1.,-3.16619526353726E-17,0.));
#8039=DIRECTION('',(1.,3.16619526353726E-17,0.));
#8040=DIRECTION('center_axis',(0.,0.,-1.));
#8041=DIRECTION('ref_axis',(1.,0.,0.));
#8042=DIRECTION('center_axis',(0.,-1.,0.));
#8043=DIRECTION('ref_axis',(0.,0.,-1.));
#8044=DIRECTION('',(0.,0.,-1.));
#8045=DIRECTION('',(-1.,0.,0.));
#8046=DIRECTION('',(0.,0.,-1.));
#8047=DIRECTION('center_axis',(0.,0.,-1.));
#8048=DIRECTION('ref_axis',(1.,1.22464679914735E-16,0.));
#8049=DIRECTION('',(0.,0.,-1.));
#8050=DIRECTION('center_axis',(0.,0.,1.));
#8051=DIRECTION('ref_axis',(1.,0.,0.));
#8052=DIRECTION('center_axis',(0.,-1.,0.));
#8053=DIRECTION('ref_axis',(0.,0.,-1.));
#8054=DIRECTION('',(0.,0.,-1.));
#8055=DIRECTION('',(-1.,0.,0.));
#8056=DIRECTION('center_axis',(1.,0.,0.));
#8057=DIRECTION('ref_axis',(0.,0.,-1.));
#8058=DIRECTION('',(0.,-1.,0.));
#8059=DIRECTION('center_axis',(0.,0.,1.));
#8060=DIRECTION('ref_axis',(1.,0.,0.));
#8061=DIRECTION('center_axis',(0.,0.,1.));
#8062=DIRECTION('ref_axis',(1.,0.,0.));
#10160=CARTESIAN_POINT('',(0.,0.,0.));
#10161=CARTESIAN_POINT('Origin',(-12.5,-8.67361737988404E-16,2.5));
#10162=CARTESIAN_POINT('',(-11.,-1.05105875786051E-15,2.5));
#10163=CARTESIAN_POINT('Origin',(-12.5,-8.67361737988404E-16,2.5));
#10164=CARTESIAN_POINT('',(-11.,-1.05105875786051E-15,0.));
#10165=CARTESIAN_POINT('',(-11.,-1.05105875786051E-15,2.5));
#10166=CARTESIAN_POINT('Origin',(-12.5,-8.67361737988404E-16,0.));
#10167=CARTESIAN_POINT('Origin',(-12.5,-8.67361737988404E-16,2.5));
#10168=CARTESIAN_POINT('',(-12.5,3.5,2.5));
#10169=CARTESIAN_POINT('',(-12.5,-3.5,2.5));
#10170=CARTESIAN_POINT('Origin',(-12.5,-8.67361737988404E-16,2.5));
#10171=CARTESIAN_POINT('',(-12.5,3.5,0.));
#10172=CARTESIAN_POINT('',(-12.5,3.5,2.5));
#10173=CARTESIAN_POINT('',(-12.5,-3.5,0.));
#10174=CARTESIAN_POINT('Origin',(-12.5,-8.67361737988404E-16,0.));
#10175=CARTESIAN_POINT('',(-12.5,-3.5,2.5));
#10176=CARTESIAN_POINT('Origin',(31.,0.,5.));
#10177=CARTESIAN_POINT('',(34.,-3.67394039744206E-16,3.));
#10178=CARTESIAN_POINT('Origin',(31.,0.,3.));
#10179=CARTESIAN_POINT('',(34.,-3.67394039744206E-16,5.));
#10180=CARTESIAN_POINT('',(34.,-3.67394039744206E-16,5.));
#10181=CARTESIAN_POINT('Origin',(31.,0.,5.));
#10182=CARTESIAN_POINT('Origin',(31.,0.,0.5));
#10183=CARTESIAN_POINT('',(29.197224362268,-3.,0.5));
#10184=CARTESIAN_POINT('',(29.197224362268,3.,0.5));
#10185=CARTESIAN_POINT('Origin',(31.,0.,0.5));
#10186=CARTESIAN_POINT('',(29.197224362268,3.,0.));
#10187=CARTESIAN_POINT('',(29.197224362268,3.,0.5));
#10188=CARTESIAN_POINT('',(29.197224362268,-3.,0.));
#10189=CARTESIAN_POINT('Origin',(31.,0.,0.));
#10190=CARTESIAN_POINT('',(29.197224362268,-3.,0.5));
#10191=CARTESIAN_POINT('Origin',(0.,0.,2.5));
#10192=CARTESIAN_POINT('',(1.80277563773199,3.,2.5));
#10193=CARTESIAN_POINT('',(1.802775637732,-3.,2.5));
#10194=CARTESIAN_POINT('Origin',(0.,0.,2.5));
#10195=CARTESIAN_POINT('',(1.80277563773199,3.,3.));
#10196=CARTESIAN_POINT('',(1.80277563773199,3.,2.5));
#10197=CARTESIAN_POINT('',(1.802775637732,-3.,3.));
#10198=CARTESIAN_POINT('Origin',(0.,0.,3.));
#10199=CARTESIAN_POINT('',(1.802775637732,-3.,2.5));
#10200=CARTESIAN_POINT('Origin',(31.,0.,3.));
#10201=CARTESIAN_POINT('',(32.5,-1.83697019872104E-16,5.));
#10202=CARTESIAN_POINT('Origin',(31.,0.,5.));
#10203=CARTESIAN_POINT('',(32.5,-1.83697019872104E-16,0.));
#10204=CARTESIAN_POINT('',(32.5,-1.83697019872104E-16,3.));
#10205=CARTESIAN_POINT('Origin',(31.,0.,0.));
#10206=CARTESIAN_POINT('Origin',(0.,0.,3.));
#10207=CARTESIAN_POINT('',(1.5,-1.83697019872103E-16,5.));
#10208=CARTESIAN_POINT('Origin',(0.,0.,5.));
#10209=CARTESIAN_POINT('',(1.5,-1.83697019872103E-16,0.));
#10210=CARTESIAN_POINT('',(1.5,-1.83697019872103E-16,3.));
#10211=CARTESIAN_POINT('Origin',(0.,0.,0.));
#10212=CARTESIAN_POINT('Origin',(0.,0.,2.5));
#10213=CARTESIAN_POINT('',(-4.,-3.5,2.5));
#10214=CARTESIAN_POINT('',(-12.5,-3.5,2.5));
#10215=CARTESIAN_POINT('',(-4.,3.5,2.5));
#10216=CARTESIAN_POINT('',(-4.,-3.5,2.5));
#10217=CARTESIAN_POINT('',(0.,3.5,2.5));
#10218=CARTESIAN_POINT('Origin',(0.,0.,3.));
#10219=CARTESIAN_POINT('',(-2.82842712474619,-1.,3.));
#10220=CARTESIAN_POINT('',(-2.82842712474619,1.,3.));
#10221=CARTESIAN_POINT('Origin',(0.,0.,3.));
#10222=CARTESIAN_POINT('',(-4.,-1.,3.));
#10223=CARTESIAN_POINT('',(0.,-1.,3.));
#10224=CARTESIAN_POINT('',(-4.,-3.5,3.));
#10225=CARTESIAN_POINT('',(-4.,-3.5,3.));
#10226=CARTESIAN_POINT('',(31.,-3.5,3.));
#10227=CARTESIAN_POINT('',(31.,-3.5,3.));
#10228=CARTESIAN_POINT('',(31.,3.5,3.));
#10229=CARTESIAN_POINT('Origin',(31.,0.,3.));
#10230=CARTESIAN_POINT('',(-4.,3.5,3.));
#10231=CARTESIAN_POINT('',(0.,3.5,3.));
#10232=CARTESIAN_POINT('',(-4.,1.,3.));
#10233=CARTESIAN_POINT('',(-4.,-3.5,3.));
#10234=CARTESIAN_POINT('',(0.,1.,3.));
#10235=CARTESIAN_POINT('',(29.197224362268,-3.,3.));
#10236=CARTESIAN_POINT('',(29.197224362268,3.,3.));
#10237=CARTESIAN_POINT('Origin',(31.,0.,3.));
#10238=CARTESIAN_POINT('',(1.802775637732,-3.,3.));
#10239=CARTESIAN_POINT('',(1.802775637732,3.,3.));
#10240=CARTESIAN_POINT('Origin',(0.,0.,0.));
#10241=CARTESIAN_POINT('',(31.,-3.5,0.));
#10242=CARTESIAN_POINT('',(31.,-3.5,0.));
#10243=CARTESIAN_POINT('',(31.,3.5,0.));
#10244=CARTESIAN_POINT('',(0.,3.5,0.));
#10245=CARTESIAN_POINT('Origin',(31.,0.,0.));
#10246=CARTESIAN_POINT('',(1.80277563773199,3.,0.));
#10247=CARTESIAN_POINT('',(1.802775637732,3.,0.));
#10248=CARTESIAN_POINT('',(1.802775637732,-3.,0.));
#10249=CARTESIAN_POINT('Origin',(0.,0.,0.));
#10250=CARTESIAN_POINT('',(1.802775637732,-3.,0.));
#10251=CARTESIAN_POINT('Origin',(31.,-3.5,3.));
#10252=CARTESIAN_POINT('',(31.,-3.5,3.));
#10253=CARTESIAN_POINT('',(-4.,-3.5,3.));
#10254=CARTESIAN_POINT('Origin',(31.,0.,3.));
#10255=CARTESIAN_POINT('',(31.,3.5,3.));
#10256=CARTESIAN_POINT('Origin',(0.,3.5,3.));
#10257=CARTESIAN_POINT('',(-4.,3.5,3.));
#10258=CARTESIAN_POINT('Origin',(31.,0.,2.5));
#10259=CARTESIAN_POINT('',(29.197224362268,3.,2.5));
#10260=CARTESIAN_POINT('',(29.197224362268,3.,2.5));
#10261=CARTESIAN_POINT('',(29.197224362268,-3.,2.5));
#10262=CARTESIAN_POINT('Origin',(31.,0.,2.5));
#10263=CARTESIAN_POINT('',(29.197224362268,-3.,2.5));
#10264=CARTESIAN_POINT('Origin',(1.802775637732,-3.,2.5));
#10265=CARTESIAN_POINT('',(1.802775637732,-3.,2.5));
#10266=CARTESIAN_POINT('Origin',(1.802775637732,3.,2.5));
#10267=CARTESIAN_POINT('',(1.802775637732,3.,2.5));
#10268=CARTESIAN_POINT('Origin',(31.,0.,2.5));
#10269=CARTESIAN_POINT('Origin',(1.802775637732,3.,0.5));
#10270=CARTESIAN_POINT('',(1.80277563773199,3.,0.5));
#10271=CARTESIAN_POINT('',(1.802775637732,3.,0.5));
#10272=CARTESIAN_POINT('',(1.80277563773199,3.,0.5));
#10273=CARTESIAN_POINT('Origin',(0.,0.,0.5));
#10274=CARTESIAN_POINT('',(1.802775637732,-3.,0.5));
#10275=CARTESIAN_POINT('Origin',(0.,0.,0.5));
#10276=CARTESIAN_POINT('',(1.802775637732,-3.,0.5));
#10277=CARTESIAN_POINT('Origin',(1.802775637732,-3.,0.5));
#10278=CARTESIAN_POINT('',(1.802775637732,-3.,0.5));
#10279=CARTESIAN_POINT('Origin',(31.,0.,0.5));
#10280=CARTESIAN_POINT('Origin',(0.,-1.,5.));
#10281=CARTESIAN_POINT('',(-2.82842712474619,-1.,5.));
#10282=CARTESIAN_POINT('',(-2.82842712474619,-1.,5.));
#10283=CARTESIAN_POINT('',(-4.,-1.,5.));
#10284=CARTESIAN_POINT('',(0.,-1.,5.));
#10285=CARTESIAN_POINT('',(-4.,-1.,5.));
#10286=CARTESIAN_POINT('Origin',(0.,0.,5.));
#10287=CARTESIAN_POINT('',(-2.82842712474619,1.,5.));
#10288=CARTESIAN_POINT('',(-2.82842712474619,1.,5.));
#10289=CARTESIAN_POINT('Origin',(0.,0.,5.));
#10290=CARTESIAN_POINT('Origin',(0.,1.,5.));
#10291=CARTESIAN_POINT('',(-4.,1.,5.));
#10292=CARTESIAN_POINT('',(-4.,1.,5.));
#10293=CARTESIAN_POINT('',(0.,1.,5.));
#10294=CARTESIAN_POINT('Origin',(-4.,0.,5.));
#10295=CARTESIAN_POINT('',(-4.,0.,5.));
#10296=CARTESIAN_POINT('Origin',(0.,0.,5.));
#10297=CARTESIAN_POINT('Origin',(0.,0.,5.));
#11915=UNCERTAINTY_MEASURE_WITH_UNIT(LENGTH_MEASURE(0.01),#11934,
'DISTANCE_ACCURACY_VALUE',
'Maximum model space distance between geometric entities at asserted c
onnectivities');
#11922=UNCERTAINTY_MEASURE_WITH_UNIT(LENGTH_MEASURE(0.01),#11934,
'DISTANCE_ACCURACY_VALUE',
'Maximum model space distance between geometric entities at asserted c
onnectivities');
#11926=(
GEOMETRIC_REPRESENTATION_CONTEXT(3)
GLOBAL_UNCERTAINTY_ASSIGNED_CONTEXT((#11915))
GLOBAL_UNIT_ASSIGNED_CONTEXT((#11934,#11936,#11937))
REPRESENTATION_CONTEXT('','3D')
);
#11933=(
GEOMETRIC_REPRESENTATION_CONTEXT(3)
GLOBAL_UNCERTAINTY_ASSIGNED_CONTEXT((#11922))
GLOBAL_UNIT_ASSIGNED_CONTEXT((#11934,#11936,#11937))
REPRESENTATION_CONTEXT('','3D')
);
#11934=(
LENGTH_UNIT()
NAMED_UNIT(*)
SI_UNIT(.MILLI.,.METRE.)
);
#11936=(
NAMED_UNIT(*)
PLANE_ANGLE_UNIT()
SI_UNIT($,.RADIAN.)
);
#11937=(
NAMED_UNIT(*)
SI_UNIT($,.STERADIAN.)
SOLID_ANGLE_UNIT()
);
#11941=SHAPE_DEFINITION_REPRESENTATION(#11951,#11990);
#11951=PRODUCT_DEFINITION_SHAPE('',$,#12001);
#11990=SHAPE_REPRESENTATION('',(#6849),#11926);
#11997=PRODUCT_DEFINITION_CONTEXT('part definition',#12029,'design');
#12001=PRODUCT_DEFINITION('Long Drive Link','Long Drive Link',#12011,#11997);
#12011=PRODUCT_DEFINITION_FORMATION('',$,#12034);
#12029=APPLICATION_CONTEXT(
'Core Data for Automotive Mechanical Design Process');
#12030=PRODUCT_CONTEXT('part definition',#12029,'mechanical');
#12034=PRODUCT('Long Drive Link','Long Drive Link',$,(#12030));
#12043=PRESENTATION_STYLE_ASSIGNMENT((#12047));
#12047=SURFACE_STYLE_USAGE(.BOTH.,#12051);
#12051=SURFACE_SIDE_STYLE('',(#12055));
#12055=SURFACE_STYLE_FILL_AREA(#12059);
#12059=FILL_AREA_STYLE('Opaque(61,176,222)',(#12063));
#12063=FILL_AREA_STYLE_COLOUR('Opaque(61,176,222)',#12067);
#12067=COLOUR_RGB('Opaque(61,176,222)',0.23921568627451,0.690196078431373,
0.870588235294118);
ENDSEC;
END-ISO-10303-21;
